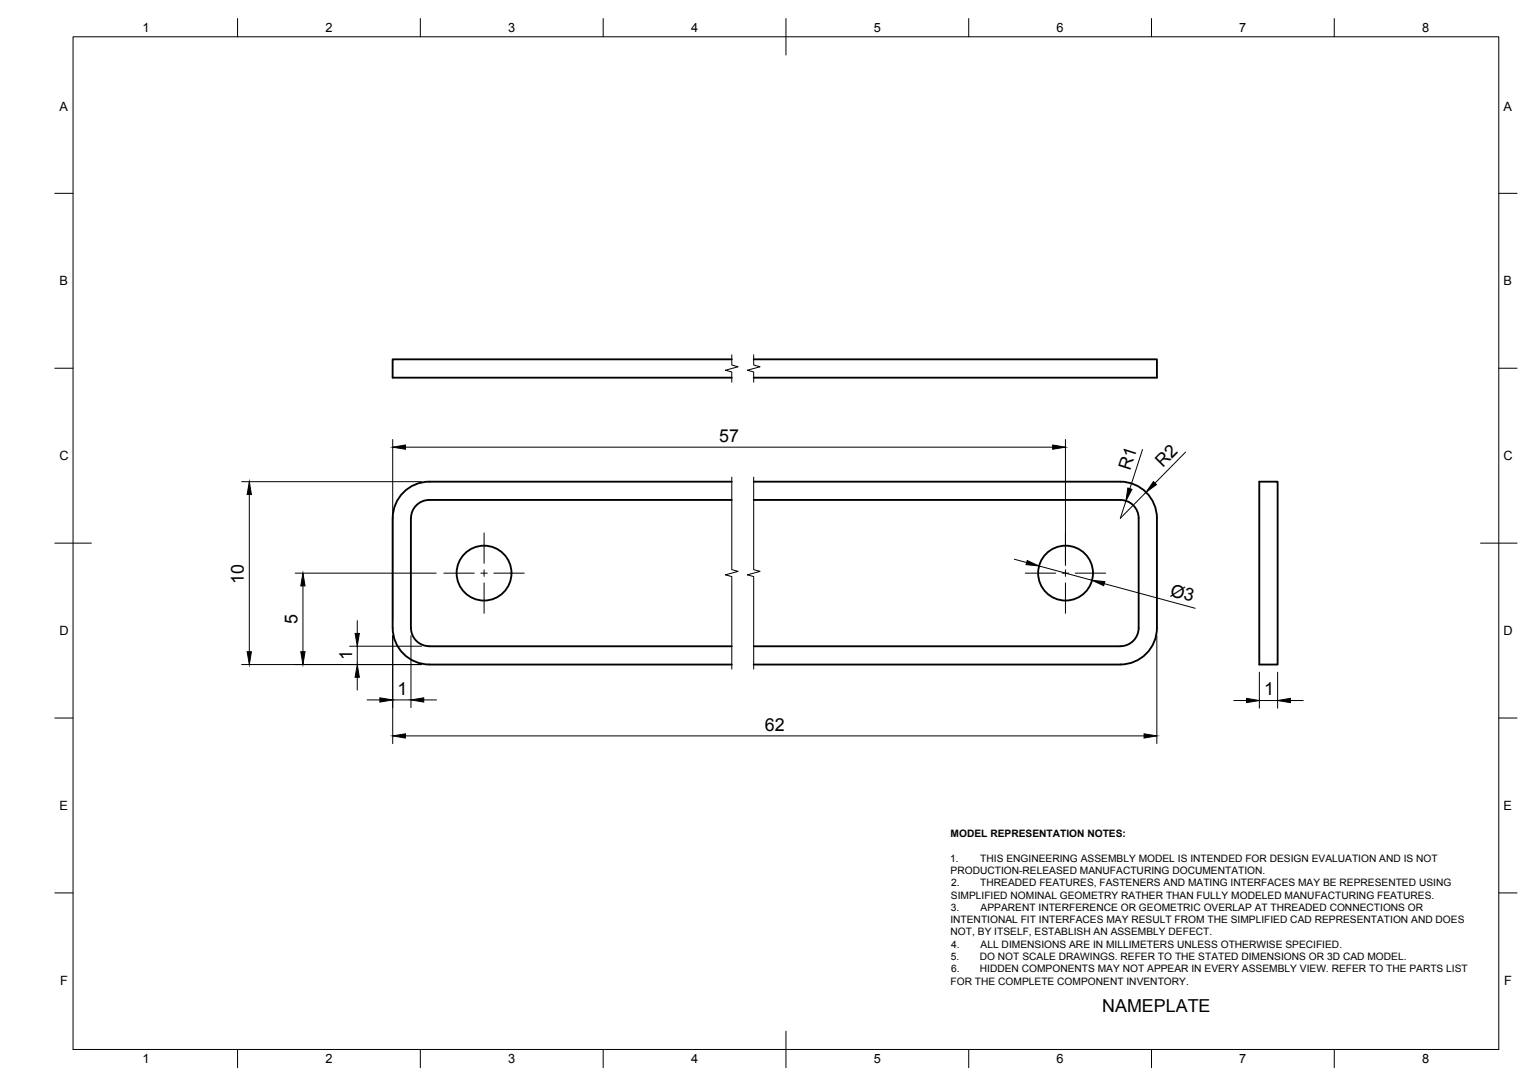
ISO-10303-21;
HEADER;
/* Generated by software containing ST-Developer
 * from STEP Tools, Inc. (www.steptools.com) 
 */

FILE_DESCRIPTION(
/* description */ (''),
/* implementation_level */ '2;1');

FILE_NAME(
/* name */ 'NAMEPLATE.step',
/* time_stamp */ '2026-10-06T01:16:10-07:00',
/* author */ (''),
/* organization */ (''),
/* preprocessor_version */ 'ST-DEVELOPER v20.2',
/* originating_system */ 'Autodesk Translation Framework v15.15.0.0',
/* authorisation */ '');

FILE_SCHEMA (('AUTOMOTIVE_DESIGN { 1 0 10303 214 3 1 1 }'));
ENDSEC;

DATA;
#10=MECHANICAL_DESIGN_GEOMETRIC_PRESENTATION_REPRESENTATION('',(#329),#17113);
#279=SHAPE_REPRESENTATION_RELATIONSHIP('SRR','None',#17205,#295);
#295=ADVANCED_BREP_SHAPE_REPRESENTATION('',(#345),#17112);
#329=STYLED_ITEM('',(#17298),#345);
#345=MANIFOLD_SOLID_BREP('Body1',#6031);
#494=CYLINDRICAL_SURFACE('',#6939,1.5);
#495=CYLINDRICAL_SURFACE('',#6947,1.);
#496=CYLINDRICAL_SURFACE('',#6957,2.);
#497=CYLINDRICAL_SURFACE('',#6959,2.);
#498=CYLINDRICAL_SURFACE('',#6961,2.);
#499=CYLINDRICAL_SURFACE('',#6963,2.);
#500=CYLINDRICAL_SURFACE('',#6966,1.);
#501=CYLINDRICAL_SURFACE('',#6968,1.);
#502=CYLINDRICAL_SURFACE('',#6970,1.);
#503=CYLINDRICAL_SURFACE('',#6972,1.5);
#631=FACE_BOUND('',#1835,.T.);
#632=FACE_BOUND('',#1836,.T.);
#633=FACE_BOUND('',#1839,.T.);
#634=FACE_BOUND('',#1840,.T.);
#635=FACE_BOUND('',#1843,.T.);
#988=CIRCLE('',#6933,2.);
#989=CIRCLE('',#6934,2.);
#990=CIRCLE('',#6935,2.);
#991=CIRCLE('',#6936,2.);
#992=CIRCLE('',#6937,1.5);
#993=CIRCLE('',#6938,1.5);
#994=CIRCLE('',#6940,1.5);
#995=CIRCLE('',#6942,1.);
#996=CIRCLE('',#6943,1.);
#997=CIRCLE('',#6944,1.);
#998=CIRCLE('',#6945,1.);
#999=CIRCLE('',#6946,1.5);
#1000=CIRCLE('',#6948,1.);
#1001=CIRCLE('',#6950,2.);
#1002=CIRCLE('',#6951,2.);
#1003=CIRCLE('',#6952,2.);
#1004=CIRCLE('',#6953,2.);
#1005=CIRCLE('',#6954,1.);
#1006=CIRCLE('',#6955,1.);
#1007=CIRCLE('',#6956,1.);
#1347=FACE_OUTER_BOUND('',#1834,.T.);
#1348=FACE_OUTER_BOUND('',#1837,.T.);
#1349=FACE_OUTER_BOUND('',#1838,.T.);
#1350=FACE_OUTER_BOUND('',#1841,.T.);
#1351=FACE_OUTER_BOUND('',#1842,.T.);
#1352=FACE_OUTER_BOUND('',#1844,.T.);
#1353=FACE_OUTER_BOUND('',#1845,.T.);
#1354=FACE_OUTER_BOUND('',#1846,.T.);
#1355=FACE_OUTER_BOUND('',#1847,.T.);
#1356=FACE_OUTER_BOUND('',#1848,.T.);
#1357=FACE_OUTER_BOUND('',#1849,.T.);
#1358=FACE_OUTER_BOUND('',#1850,.T.);
#1359=FACE_OUTER_BOUND('',#1851,.T.);
#1360=FACE_OUTER_BOUND('',#1852,.T.);
#1361=FACE_OUTER_BOUND('',#1853,.T.);
#1362=FACE_OUTER_BOUND('',#1854,.T.);
#1363=FACE_OUTER_BOUND('',#1855,.T.);
#1364=FACE_OUTER_BOUND('',#1856,.T.);
#1365=FACE_OUTER_BOUND('',#1857,.T.);
#1366=FACE_OUTER_BOUND('',#1858,.T.);
#1367=FACE_OUTER_BOUND('',#1859,.T.);
#1834=EDGE_LOOP('',(#5396,#5397,#5398,#5399,#5400,#5401,#5402,#5403));
#1835=EDGE_LOOP('',(#5404));
#1836=EDGE_LOOP('',(#5405));
#1837=EDGE_LOOP('',(#5406,#5407,#5408,#5409));
#1838=EDGE_LOOP('',(#5410,#5411,#5412,#5413,#5414,#5415,#5416,#5417));
#1839=EDGE_LOOP('',(#5418));
#1840=EDGE_LOOP('',(#5419));
#1841=EDGE_LOOP('',(#5420,#5421,#5422,#5423));
#1842=EDGE_LOOP('',(#5424,#5425,#5426,#5427,#5428,#5429,#5430,#5431));
#1843=EDGE_LOOP('',(#5432,#5433,#5434,#5435,#5436,#5437,#5438,#5439));
#1844=EDGE_LOOP('',(#5440,#5441,#5442,#5443));
#1845=EDGE_LOOP('',(#5444,#5445,#5446,#5447));
#1846=EDGE_LOOP('',(#5448,#5449,#5450,#5451));
#1847=EDGE_LOOP('',(#5452,#5453,#5454,#5455));
#1848=EDGE_LOOP('',(#5456,#5457,#5458,#5459));
#1849=EDGE_LOOP('',(#5460,#5461,#5462,#5463));
#1850=EDGE_LOOP('',(#5464,#5465,#5466,#5467));
#1851=EDGE_LOOP('',(#5468,#5469,#5470,#5471));
#1852=EDGE_LOOP('',(#5472,#5473,#5474,#5475));
#1853=EDGE_LOOP('',(#5476,#5477,#5478,#5479));
#1854=EDGE_LOOP('',(#5480,#5481,#5482,#5483));
#1855=EDGE_LOOP('',(#5484,#5485,#5486,#5487));
#1856=EDGE_LOOP('',(#5488,#5489,#5490,#5491));
#1857=EDGE_LOOP('',(#5492,#5493,#5494,#5495));
#1858=EDGE_LOOP('',(#5496,#5497,#5498,#5499));
#1859=EDGE_LOOP('',(#5500,#5501,#5502,#5503));
#2187=LINE('',#16957,#2548);
#2188=LINE('',#16961,#2549);
#2189=LINE('',#16965,#2550);
#2190=LINE('',#16968,#2551);
#2191=LINE('',#16975,#2552);
#2192=LINE('',#16982,#2553);
#2193=LINE('',#16986,#2554);
#2194=LINE('',#16990,#2555);
#2195=LINE('',#16993,#2556);
#2196=LINE('',#17000,#2557);
#2197=LINE('',#17001,#2558);
#2198=LINE('',#17007,#2559);
#2199=LINE('',#17011,#2560);
#2200=LINE('',#17015,#2561);
#2201=LINE('',#17018,#2562);
#2202=LINE('',#17020,#2563);
#2203=LINE('',#17024,#2564);
#2204=LINE('',#17028,#2565);
#2205=LINE('',#17031,#2566);
#2206=LINE('',#17033,#2567);
#2207=LINE('',#17034,#2568);
#2208=LINE('',#17036,#2569);
#2209=LINE('',#17038,#2570);
#2210=LINE('',#17040,#2571);
#2211=LINE('',#17042,#2572);
#2212=LINE('',#17044,#2573);
#2213=LINE('',#17046,#2574);
#2214=LINE('',#17049,#2575);
#2215=LINE('',#17051,#2576);
#2216=LINE('',#17053,#2577);
#2217=LINE('',#17055,#2578);
#2218=LINE('',#17057,#2579);
#2219=LINE('',#17059,#2580);
#2220=LINE('',#17062,#2581);
#2548=VECTOR('',#8755,58.);
#2549=VECTOR('',#8758,6.);
#2550=VECTOR('',#8761,58.);
#2551=VECTOR('',#8764,6.);
#2552=VECTOR('',#8771,1.5);
#2553=VECTOR('',#8778,6.);
#2554=VECTOR('',#8781,58.);
#2555=VECTOR('',#8784,6.);
#2556=VECTOR('',#8787,58.);
#2557=VECTOR('',#8794,0.5);
#2558=VECTOR('',#8795,0.5);
#2559=VECTOR('',#8800,6.);
#2560=VECTOR('',#8803,58.);
#2561=VECTOR('',#8806,6.);
#2562=VECTOR('',#8809,58.);
#2563=VECTOR('',#8810,58.);
#2564=VECTOR('',#8813,6.);
#2565=VECTOR('',#8816,58.);
#2566=VECTOR('',#8819,6.);
#2567=VECTOR('',#8822,1.);
#2568=VECTOR('',#8823,1.);
#2569=VECTOR('',#8826,1.);
#2570=VECTOR('',#8829,1.);
#2571=VECTOR('',#8832,1.);
#2572=VECTOR('',#8835,1.);
#2573=VECTOR('',#8838,1.);
#2574=VECTOR('',#8841,1.);
#2575=VECTOR('',#8846,0.5);
#2576=VECTOR('',#8849,0.5);
#2577=VECTOR('',#8852,0.5);
#2578=VECTOR('',#8855,0.5);
#2579=VECTOR('',#8858,0.5);
#2580=VECTOR('',#8861,0.5);
#2581=VECTOR('',#8866,1.5);
#3068=VERTEX_POINT('',#16953);
#3069=VERTEX_POINT('',#16954);
#3070=VERTEX_POINT('',#16956);
#3071=VERTEX_POINT('',#16958);
#3072=VERTEX_POINT('',#16960);
#3073=VERTEX_POINT('',#16962);
#3074=VERTEX_POINT('',#16964);
#3075=VERTEX_POINT('',#16966);
#3076=VERTEX_POINT('',#16969);
#3077=VERTEX_POINT('',#16971);
#3078=VERTEX_POINT('',#16974);
#3079=VERTEX_POINT('',#16978);
#3080=VERTEX_POINT('',#16979);
#3081=VERTEX_POINT('',#16981);
#3082=VERTEX_POINT('',#16983);
#3083=VERTEX_POINT('',#16985);
#3084=VERTEX_POINT('',#16987);
#3085=VERTEX_POINT('',#16989);
#3086=VERTEX_POINT('',#16991);
#3087=VERTEX_POINT('',#16994);
#3088=VERTEX_POINT('',#16997);
#3089=VERTEX_POINT('',#16998);
#3090=VERTEX_POINT('',#17003);
#3091=VERTEX_POINT('',#17004);
#3092=VERTEX_POINT('',#17006);
#3093=VERTEX_POINT('',#17008);
#3094=VERTEX_POINT('',#17010);
#3095=VERTEX_POINT('',#17012);
#3096=VERTEX_POINT('',#17014);
#3097=VERTEX_POINT('',#17016);
#3098=VERTEX_POINT('',#17019);
#3099=VERTEX_POINT('',#17021);
#3100=VERTEX_POINT('',#17023);
#3101=VERTEX_POINT('',#17025);
#3102=VERTEX_POINT('',#17027);
#3103=VERTEX_POINT('',#17029);
#3862=EDGE_CURVE('',#3068,#3069,#988,.T.);
#3863=EDGE_CURVE('',#3070,#3068,#2187,.T.);
#3864=EDGE_CURVE('',#3071,#3070,#989,.T.);
#3865=EDGE_CURVE('',#3072,#3071,#2188,.T.);
#3866=EDGE_CURVE('',#3073,#3072,#990,.T.);
#3867=EDGE_CURVE('',#3074,#3073,#2189,.T.);
#3868=EDGE_CURVE('',#3075,#3074,#991,.T.);
#3869=EDGE_CURVE('',#3069,#3075,#2190,.T.);
#3870=EDGE_CURVE('',#3076,#3076,#992,.T.);
#3871=EDGE_CURVE('',#3077,#3077,#993,.T.);
#3872=EDGE_CURVE('',#3077,#3078,#2191,.T.);
#3873=EDGE_CURVE('',#3078,#3078,#994,.T.);
#3874=EDGE_CURVE('',#3079,#3080,#995,.T.);
#3875=EDGE_CURVE('',#3080,#3081,#2192,.T.);
#3876=EDGE_CURVE('',#3081,#3082,#996,.T.);
#3877=EDGE_CURVE('',#3082,#3083,#2193,.T.);
#3878=EDGE_CURVE('',#3083,#3084,#997,.T.);
#3879=EDGE_CURVE('',#3084,#3085,#2194,.T.);
#3880=EDGE_CURVE('',#3085,#3086,#998,.T.);
#3881=EDGE_CURVE('',#3086,#3079,#2195,.T.);
#3882=EDGE_CURVE('',#3087,#3087,#999,.T.);
#3883=EDGE_CURVE('',#3088,#3089,#1000,.T.);
#3884=EDGE_CURVE('',#3089,#3080,#2196,.T.);
#3885=EDGE_CURVE('',#3088,#3079,#2197,.T.);
#3886=EDGE_CURVE('',#3090,#3091,#1001,.T.);
#3887=EDGE_CURVE('',#3091,#3092,#2198,.T.);
#3888=EDGE_CURVE('',#3092,#3093,#1002,.T.);
#3889=EDGE_CURVE('',#3093,#3094,#2199,.T.);
#3890=EDGE_CURVE('',#3094,#3095,#1003,.T.);
#3891=EDGE_CURVE('',#3095,#3096,#2200,.T.);
#3892=EDGE_CURVE('',#3096,#3097,#1004,.T.);
#3893=EDGE_CURVE('',#3097,#3090,#2201,.T.);
#3894=EDGE_CURVE('',#3098,#3088,#2202,.T.);
#3895=EDGE_CURVE('',#3099,#3098,#1005,.T.);
#3896=EDGE_CURVE('',#3100,#3099,#2203,.T.);
#3897=EDGE_CURVE('',#3101,#3100,#1006,.T.);
#3898=EDGE_CURVE('',#3102,#3101,#2204,.T.);
#3899=EDGE_CURVE('',#3103,#3102,#1007,.T.);
#3900=EDGE_CURVE('',#3089,#3103,#2205,.T.);
#3901=EDGE_CURVE('',#3069,#3091,#2206,.T.);
#3902=EDGE_CURVE('',#3068,#3090,#2207,.T.);
#3903=EDGE_CURVE('',#3070,#3097,#2208,.T.);
#3904=EDGE_CURVE('',#3071,#3096,#2209,.T.);
#3905=EDGE_CURVE('',#3072,#3095,#2210,.T.);
#3906=EDGE_CURVE('',#3073,#3094,#2211,.T.);
#3907=EDGE_CURVE('',#3074,#3093,#2212,.T.);
#3908=EDGE_CURVE('',#3075,#3092,#2213,.T.);
#3909=EDGE_CURVE('',#3103,#3081,#2214,.T.);
#3910=EDGE_CURVE('',#3102,#3082,#2215,.T.);
#3911=EDGE_CURVE('',#3101,#3083,#2216,.T.);
#3912=EDGE_CURVE('',#3100,#3084,#2217,.T.);
#3913=EDGE_CURVE('',#3099,#3085,#2218,.T.);
#3914=EDGE_CURVE('',#3098,#3086,#2219,.T.);
#3915=EDGE_CURVE('',#3076,#3087,#2220,.T.);
#5396=ORIENTED_EDGE('',*,*,#3862,.F.);
#5397=ORIENTED_EDGE('',*,*,#3863,.F.);
#5398=ORIENTED_EDGE('',*,*,#3864,.F.);
#5399=ORIENTED_EDGE('',*,*,#3865,.F.);
#5400=ORIENTED_EDGE('',*,*,#3866,.F.);
#5401=ORIENTED_EDGE('',*,*,#3867,.F.);
#5402=ORIENTED_EDGE('',*,*,#3868,.F.);
#5403=ORIENTED_EDGE('',*,*,#3869,.F.);
#5404=ORIENTED_EDGE('',*,*,#3870,.F.);
#5405=ORIENTED_EDGE('',*,*,#3871,.F.);
#5406=ORIENTED_EDGE('',*,*,#3871,.T.);
#5407=ORIENTED_EDGE('',*,*,#3872,.T.);
#5408=ORIENTED_EDGE('',*,*,#3873,.T.);
#5409=ORIENTED_EDGE('',*,*,#3872,.F.);
#5410=ORIENTED_EDGE('',*,*,#3874,.T.);
#5411=ORIENTED_EDGE('',*,*,#3875,.T.);
#5412=ORIENTED_EDGE('',*,*,#3876,.T.);
#5413=ORIENTED_EDGE('',*,*,#3877,.T.);
#5414=ORIENTED_EDGE('',*,*,#3878,.T.);
#5415=ORIENTED_EDGE('',*,*,#3879,.T.);
#5416=ORIENTED_EDGE('',*,*,#3880,.T.);
#5417=ORIENTED_EDGE('',*,*,#3881,.T.);
#5418=ORIENTED_EDGE('',*,*,#3873,.F.);
#5419=ORIENTED_EDGE('',*,*,#3882,.F.);
#5420=ORIENTED_EDGE('',*,*,#3883,.T.);
#5421=ORIENTED_EDGE('',*,*,#3884,.T.);
#5422=ORIENTED_EDGE('',*,*,#3874,.F.);
#5423=ORIENTED_EDGE('',*,*,#3885,.F.);
#5424=ORIENTED_EDGE('',*,*,#3886,.T.);
#5425=ORIENTED_EDGE('',*,*,#3887,.T.);
#5426=ORIENTED_EDGE('',*,*,#3888,.T.);
#5427=ORIENTED_EDGE('',*,*,#3889,.T.);
#5428=ORIENTED_EDGE('',*,*,#3890,.T.);
#5429=ORIENTED_EDGE('',*,*,#3891,.T.);
#5430=ORIENTED_EDGE('',*,*,#3892,.T.);
#5431=ORIENTED_EDGE('',*,*,#3893,.T.);
#5432=ORIENTED_EDGE('',*,*,#3883,.F.);
#5433=ORIENTED_EDGE('',*,*,#3894,.F.);
#5434=ORIENTED_EDGE('',*,*,#3895,.F.);
#5435=ORIENTED_EDGE('',*,*,#3896,.F.);
#5436=ORIENTED_EDGE('',*,*,#3897,.F.);
#5437=ORIENTED_EDGE('',*,*,#3898,.F.);
#5438=ORIENTED_EDGE('',*,*,#3899,.F.);
#5439=ORIENTED_EDGE('',*,*,#3900,.F.);
#5440=ORIENTED_EDGE('',*,*,#3862,.T.);
#5441=ORIENTED_EDGE('',*,*,#3901,.T.);
#5442=ORIENTED_EDGE('',*,*,#3886,.F.);
#5443=ORIENTED_EDGE('',*,*,#3902,.F.);
#5444=ORIENTED_EDGE('',*,*,#3863,.T.);
#5445=ORIENTED_EDGE('',*,*,#3902,.T.);
#5446=ORIENTED_EDGE('',*,*,#3893,.F.);
#5447=ORIENTED_EDGE('',*,*,#3903,.F.);
#5448=ORIENTED_EDGE('',*,*,#3864,.T.);
#5449=ORIENTED_EDGE('',*,*,#3903,.T.);
#5450=ORIENTED_EDGE('',*,*,#3892,.F.);
#5451=ORIENTED_EDGE('',*,*,#3904,.F.);
#5452=ORIENTED_EDGE('',*,*,#3865,.T.);
#5453=ORIENTED_EDGE('',*,*,#3904,.T.);
#5454=ORIENTED_EDGE('',*,*,#3891,.F.);
#5455=ORIENTED_EDGE('',*,*,#3905,.F.);
#5456=ORIENTED_EDGE('',*,*,#3866,.T.);
#5457=ORIENTED_EDGE('',*,*,#3905,.T.);
#5458=ORIENTED_EDGE('',*,*,#3890,.F.);
#5459=ORIENTED_EDGE('',*,*,#3906,.F.);
#5460=ORIENTED_EDGE('',*,*,#3867,.T.);
#5461=ORIENTED_EDGE('',*,*,#3906,.T.);
#5462=ORIENTED_EDGE('',*,*,#3889,.F.);
#5463=ORIENTED_EDGE('',*,*,#3907,.F.);
#5464=ORIENTED_EDGE('',*,*,#3868,.T.);
#5465=ORIENTED_EDGE('',*,*,#3907,.T.);
#5466=ORIENTED_EDGE('',*,*,#3888,.F.);
#5467=ORIENTED_EDGE('',*,*,#3908,.F.);
#5468=ORIENTED_EDGE('',*,*,#3869,.T.);
#5469=ORIENTED_EDGE('',*,*,#3908,.T.);
#5470=ORIENTED_EDGE('',*,*,#3887,.F.);
#5471=ORIENTED_EDGE('',*,*,#3901,.F.);
#5472=ORIENTED_EDGE('',*,*,#3900,.T.);
#5473=ORIENTED_EDGE('',*,*,#3909,.T.);
#5474=ORIENTED_EDGE('',*,*,#3875,.F.);
#5475=ORIENTED_EDGE('',*,*,#3884,.F.);
#5476=ORIENTED_EDGE('',*,*,#3899,.T.);
#5477=ORIENTED_EDGE('',*,*,#3910,.T.);
#5478=ORIENTED_EDGE('',*,*,#3876,.F.);
#5479=ORIENTED_EDGE('',*,*,#3909,.F.);
#5480=ORIENTED_EDGE('',*,*,#3898,.T.);
#5481=ORIENTED_EDGE('',*,*,#3911,.T.);
#5482=ORIENTED_EDGE('',*,*,#3877,.F.);
#5483=ORIENTED_EDGE('',*,*,#3910,.F.);
#5484=ORIENTED_EDGE('',*,*,#3897,.T.);
#5485=ORIENTED_EDGE('',*,*,#3912,.T.);
#5486=ORIENTED_EDGE('',*,*,#3878,.F.);
#5487=ORIENTED_EDGE('',*,*,#3911,.F.);
#5488=ORIENTED_EDGE('',*,*,#3896,.T.);
#5489=ORIENTED_EDGE('',*,*,#3913,.T.);
#5490=ORIENTED_EDGE('',*,*,#3879,.F.);
#5491=ORIENTED_EDGE('',*,*,#3912,.F.);
#5492=ORIENTED_EDGE('',*,*,#3895,.T.);
#5493=ORIENTED_EDGE('',*,*,#3914,.T.);
#5494=ORIENTED_EDGE('',*,*,#3880,.F.);
#5495=ORIENTED_EDGE('',*,*,#3913,.F.);
#5496=ORIENTED_EDGE('',*,*,#3894,.T.);
#5497=ORIENTED_EDGE('',*,*,#3885,.T.);
#5498=ORIENTED_EDGE('',*,*,#3881,.F.);
#5499=ORIENTED_EDGE('',*,*,#3914,.F.);
#5500=ORIENTED_EDGE('',*,*,#3870,.T.);
#5501=ORIENTED_EDGE('',*,*,#3915,.T.);
#5502=ORIENTED_EDGE('',*,*,#3882,.T.);
#5503=ORIENTED_EDGE('',*,*,#3915,.F.);
#5645=PLANE('',#6932);
#5646=PLANE('',#6941);
#5647=PLANE('',#6949);
#5648=PLANE('',#6958);
#5649=PLANE('',#6960);
#5650=PLANE('',#6962);
#5651=PLANE('',#6964);
#5652=PLANE('',#6965);
#5653=PLANE('',#6967);
#5654=PLANE('',#6969);
#5655=PLANE('',#6971);
#5995=ADVANCED_FACE('',(#1347,#631,#632),#5645,.F.);
#5996=ADVANCED_FACE('',(#1348),#494,.F.);
#5997=ADVANCED_FACE('',(#1349,#633,#634),#5646,.T.);
#5998=ADVANCED_FACE('',(#1350),#495,.F.);
#5999=ADVANCED_FACE('',(#1351,#635),#5647,.T.);
#6000=ADVANCED_FACE('',(#1352),#496,.T.);
#6001=ADVANCED_FACE('',(#1353),#5648,.T.);
#6002=ADVANCED_FACE('',(#1354),#497,.T.);
#6003=ADVANCED_FACE('',(#1355),#5649,.T.);
#6004=ADVANCED_FACE('',(#1356),#498,.T.);
#6005=ADVANCED_FACE('',(#1357),#5650,.T.);
#6006=ADVANCED_FACE('',(#1358),#499,.T.);
#6007=ADVANCED_FACE('',(#1359),#5651,.T.);
#6008=ADVANCED_FACE('',(#1360),#5652,.F.);
#6009=ADVANCED_FACE('',(#1361),#500,.F.);
#6010=ADVANCED_FACE('',(#1362),#5653,.F.);
#6011=ADVANCED_FACE('',(#1363),#501,.F.);
#6012=ADVANCED_FACE('',(#1364),#5654,.F.);
#6013=ADVANCED_FACE('',(#1365),#502,.F.);
#6014=ADVANCED_FACE('',(#1366),#5655,.F.);
#6015=ADVANCED_FACE('',(#1367),#503,.F.);
#6031=CLOSED_SHELL('',(#5995,#5996,#5997,#5998,#5999,#6000,#6001,#6002,
#6003,#6004,#6005,#6006,#6007,#6008,#6009,#6010,#6011,#6012,#6013,#6014,
#6015));
#6931=AXIS2_PLACEMENT_3D('',#16951,#8749,#8750);
#6932=AXIS2_PLACEMENT_3D('',#16952,#8751,#8752);
#6933=AXIS2_PLACEMENT_3D('',#16955,#8753,#8754);
#6934=AXIS2_PLACEMENT_3D('',#16959,#8756,#8757);
#6935=AXIS2_PLACEMENT_3D('',#16963,#8759,#8760);
#6936=AXIS2_PLACEMENT_3D('',#16967,#8762,#8763);
#6937=AXIS2_PLACEMENT_3D('',#16970,#8765,#8766);
#6938=AXIS2_PLACEMENT_3D('',#16972,#8767,#8768);
#6939=AXIS2_PLACEMENT_3D('',#16973,#8769,#8770);
#6940=AXIS2_PLACEMENT_3D('',#16976,#8772,#8773);
#6941=AXIS2_PLACEMENT_3D('',#16977,#8774,#8775);
#6942=AXIS2_PLACEMENT_3D('',#16980,#8776,#8777);
#6943=AXIS2_PLACEMENT_3D('',#16984,#8779,#8780);
#6944=AXIS2_PLACEMENT_3D('',#16988,#8782,#8783);
#6945=AXIS2_PLACEMENT_3D('',#16992,#8785,#8786);
#6946=AXIS2_PLACEMENT_3D('',#16995,#8788,#8789);
#6947=AXIS2_PLACEMENT_3D('',#16996,#8790,#8791);
#6948=AXIS2_PLACEMENT_3D('',#16999,#8792,#8793);
#6949=AXIS2_PLACEMENT_3D('',#17002,#8796,#8797);
#6950=AXIS2_PLACEMENT_3D('',#17005,#8798,#8799);
#6951=AXIS2_PLACEMENT_3D('',#17009,#8801,#8802);
#6952=AXIS2_PLACEMENT_3D('',#17013,#8804,#8805);
#6953=AXIS2_PLACEMENT_3D('',#17017,#8807,#8808);
#6954=AXIS2_PLACEMENT_3D('',#17022,#8811,#8812);
#6955=AXIS2_PLACEMENT_3D('',#17026,#8814,#8815);
#6956=AXIS2_PLACEMENT_3D('',#17030,#8817,#8818);
#6957=AXIS2_PLACEMENT_3D('',#17032,#8820,#8821);
#6958=AXIS2_PLACEMENT_3D('',#17035,#8824,#8825);
#6959=AXIS2_PLACEMENT_3D('',#17037,#8827,#8828);
#6960=AXIS2_PLACEMENT_3D('',#17039,#8830,#8831);
#6961=AXIS2_PLACEMENT_3D('',#17041,#8833,#8834);
#6962=AXIS2_PLACEMENT_3D('',#17043,#8836,#8837);
#6963=AXIS2_PLACEMENT_3D('',#17045,#8839,#8840);
#6964=AXIS2_PLACEMENT_3D('',#17047,#8842,#8843);
#6965=AXIS2_PLACEMENT_3D('',#17048,#8844,#8845);
#6966=AXIS2_PLACEMENT_3D('',#17050,#8847,#8848);
#6967=AXIS2_PLACEMENT_3D('',#17052,#8850,#8851);
#6968=AXIS2_PLACEMENT_3D('',#17054,#8853,#8854);
#6969=AXIS2_PLACEMENT_3D('',#17056,#8856,#8857);
#6970=AXIS2_PLACEMENT_3D('',#17058,#8859,#8860);
#6971=AXIS2_PLACEMENT_3D('',#17060,#8862,#8863);
#6972=AXIS2_PLACEMENT_3D('',#17061,#8864,#8865);
#8749=DIRECTION('axis',(0.,0.,1.));
#8750=DIRECTION('refdir',(1.,0.,0.));
#8751=DIRECTION('center_axis',(0.,0.,1.));
#8752=DIRECTION('ref_axis',(1.,0.,0.));
#8753=DIRECTION('center_axis',(0.,0.,1.));
#8754=DIRECTION('ref_axis',(0.,1.,0.));
#8755=DIRECTION('',(-1.,0.,0.));
#8756=DIRECTION('center_axis',(0.,0.,1.));
#8757=DIRECTION('ref_axis',(1.,0.,0.));
#8758=DIRECTION('',(0.,1.,0.));
#8759=DIRECTION('center_axis',(0.,0.,1.));
#8760=DIRECTION('ref_axis',(0.,-1.,0.));
#8761=DIRECTION('',(1.,0.,0.));
#8762=DIRECTION('center_axis',(0.,0.,1.));
#8763=DIRECTION('ref_axis',(-1.,0.,0.));
#8764=DIRECTION('',(0.,-1.,0.));
#8765=DIRECTION('center_axis',(0.,0.,-1.));
#8766=DIRECTION('ref_axis',(1.,0.,0.));
#8767=DIRECTION('center_axis',(0.,0.,-1.));
#8768=DIRECTION('ref_axis',(1.,0.,0.));
#8769=DIRECTION('center_axis',(0.,0.,1.));
#8770=DIRECTION('ref_axis',(1.,0.,0.));
#8771=DIRECTION('',(0.,0.,1.));
#8772=DIRECTION('center_axis',(0.,0.,1.));
#8773=DIRECTION('ref_axis',(-1.,0.,0.));
#8774=DIRECTION('center_axis',(0.,0.,1.));
#8775=DIRECTION('ref_axis',(1.,0.,0.));
#8776=DIRECTION('center_axis',(0.,0.,1.));
#8777=DIRECTION('ref_axis',(0.,1.,0.));
#8778=DIRECTION('',(0.,-1.,0.));
#8779=DIRECTION('center_axis',(0.,0.,1.));
#8780=DIRECTION('ref_axis',(-1.,0.,0.));
#8781=DIRECTION('',(1.,0.,0.));
#8782=DIRECTION('center_axis',(0.,0.,1.));
#8783=DIRECTION('ref_axis',(0.,-1.,0.));
#8784=DIRECTION('',(0.,1.,0.));
#8785=DIRECTION('center_axis',(0.,0.,1.));
#8786=DIRECTION('ref_axis',(1.,0.,0.));
#8787=DIRECTION('',(-1.,0.,0.));
#8788=DIRECTION('center_axis',(0.,0.,1.));
#8789=DIRECTION('ref_axis',(-1.,0.,0.));
#8790=DIRECTION('center_axis',(0.,0.,1.));
#8791=DIRECTION('ref_axis',(1.,0.,0.));
#8792=DIRECTION('center_axis',(0.,0.,1.));
#8793=DIRECTION('ref_axis',(0.,1.,0.));
#8794=DIRECTION('',(0.,0.,-1.));
#8795=DIRECTION('',(0.,0.,-1.));
#8796=DIRECTION('center_axis',(0.,0.,1.));
#8797=DIRECTION('ref_axis',(1.,0.,0.));
#8798=DIRECTION('center_axis',(0.,0.,1.));
#8799=DIRECTION('ref_axis',(0.,1.,0.));
#8800=DIRECTION('',(0.,-1.,0.));
#8801=DIRECTION('center_axis',(0.,0.,1.));
#8802=DIRECTION('ref_axis',(-1.,0.,0.));
#8803=DIRECTION('',(1.,0.,0.));
#8804=DIRECTION('center_axis',(0.,0.,1.));
#8805=DIRECTION('ref_axis',(0.,-1.,0.));
#8806=DIRECTION('',(0.,1.,0.));
#8807=DIRECTION('center_axis',(0.,0.,1.));
#8808=DIRECTION('ref_axis',(1.,0.,0.));
#8809=DIRECTION('',(-1.,0.,0.));
#8810=DIRECTION('',(-1.,0.,0.));
#8811=DIRECTION('center_axis',(0.,0.,1.));
#8812=DIRECTION('ref_axis',(1.,0.,0.));
#8813=DIRECTION('',(0.,1.,0.));
#8814=DIRECTION('center_axis',(0.,0.,1.));
#8815=DIRECTION('ref_axis',(0.,-1.,0.));
#8816=DIRECTION('',(1.,0.,0.));
#8817=DIRECTION('center_axis',(0.,0.,1.));
#8818=DIRECTION('ref_axis',(-1.,0.,0.));
#8819=DIRECTION('',(0.,-1.,0.));
#8820=DIRECTION('center_axis',(0.,0.,1.));
#8821=DIRECTION('ref_axis',(1.,0.,0.));
#8822=DIRECTION('',(0.,0.,1.));
#8823=DIRECTION('',(0.,0.,1.));
#8824=DIRECTION('center_axis',(0.,1.,0.));
#8825=DIRECTION('ref_axis',(-1.,0.,0.));
#8826=DIRECTION('',(0.,0.,1.));
#8827=DIRECTION('center_axis',(0.,0.,1.));
#8828=DIRECTION('ref_axis',(1.,0.,0.));
#8829=DIRECTION('',(0.,0.,1.));
#8830=DIRECTION('center_axis',(1.,0.,0.));
#8831=DIRECTION('ref_axis',(0.,1.,0.));
#8832=DIRECTION('',(0.,0.,1.));
#8833=DIRECTION('center_axis',(0.,0.,1.));
#8834=DIRECTION('ref_axis',(1.,0.,0.));
#8835=DIRECTION('',(0.,0.,1.));
#8836=DIRECTION('center_axis',(0.,-1.,0.));
#8837=DIRECTION('ref_axis',(1.,0.,0.));
#8838=DIRECTION('',(0.,0.,1.));
#8839=DIRECTION('center_axis',(0.,0.,1.));
#8840=DIRECTION('ref_axis',(1.,0.,0.));
#8841=DIRECTION('',(0.,0.,1.));
#8842=DIRECTION('center_axis',(-1.,0.,0.));
#8843=DIRECTION('ref_axis',(0.,-1.,0.));
#8844=DIRECTION('center_axis',(-1.,0.,0.));
#8845=DIRECTION('ref_axis',(0.,-1.,0.));
#8846=DIRECTION('',(0.,0.,-1.));
#8847=DIRECTION('center_axis',(0.,0.,1.));
#8848=DIRECTION('ref_axis',(1.,0.,0.));
#8849=DIRECTION('',(0.,0.,-1.));
#8850=DIRECTION('center_axis',(0.,-1.,0.));
#8851=DIRECTION('ref_axis',(1.,0.,0.));
#8852=DIRECTION('',(0.,0.,-1.));
#8853=DIRECTION('center_axis',(0.,0.,1.));
#8854=DIRECTION('ref_axis',(1.,0.,0.));
#8855=DIRECTION('',(0.,0.,-1.));
#8856=DIRECTION('center_axis',(1.,0.,0.));
#8857=DIRECTION('ref_axis',(0.,1.,0.));
#8858=DIRECTION('',(0.,0.,-1.));
#8859=DIRECTION('center_axis',(0.,0.,1.));
#8860=DIRECTION('ref_axis',(1.,0.,0.));
#8861=DIRECTION('',(0.,0.,-1.));
#8862=DIRECTION('center_axis',(0.,1.,0.));
#8863=DIRECTION('ref_axis',(-1.,0.,0.));
#8864=DIRECTION('center_axis',(0.,0.,1.));
#8865=DIRECTION('ref_axis',(1.,0.,0.));
#8866=DIRECTION('',(0.,0.,1.));
#16951=CARTESIAN_POINT('',(0.,0.,0.));
#16952=CARTESIAN_POINT('Origin',(0.,0.,-0.5));
#16953=CARTESIAN_POINT('',(-29.,5.,-0.5));
#16954=CARTESIAN_POINT('',(-31.,3.,-0.5));
#16955=CARTESIAN_POINT('Origin',(-29.,3.,-0.5));
#16956=CARTESIAN_POINT('',(29.,5.,-0.5));
#16957=CARTESIAN_POINT('',(29.,5.,-0.5));
#16958=CARTESIAN_POINT('',(31.,3.,-0.5));
#16959=CARTESIAN_POINT('Origin',(29.,3.,-0.5));
#16960=CARTESIAN_POINT('',(31.,-3.,-0.5));
#16961=CARTESIAN_POINT('',(31.,-3.,-0.5));
#16962=CARTESIAN_POINT('',(29.,-5.,-0.5));
#16963=CARTESIAN_POINT('Origin',(29.,-3.,-0.5));
#16964=CARTESIAN_POINT('',(-29.,-5.,-0.5));
#16965=CARTESIAN_POINT('',(-29.,-5.,-0.5));
#16966=CARTESIAN_POINT('',(-31.,-3.,-0.5));
#16967=CARTESIAN_POINT('Origin',(-29.,-3.,-0.5));
#16968=CARTESIAN_POINT('',(-31.,3.,-0.5));
#16969=CARTESIAN_POINT('',(24.5,0.,-0.5));
#16970=CARTESIAN_POINT('Origin',(26.,0.,-0.5));
#16971=CARTESIAN_POINT('',(-27.5,0.,-0.5));
#16972=CARTESIAN_POINT('Origin',(-26.,0.,-0.5));
#16973=CARTESIAN_POINT('Origin',(-26.,0.,-0.5));
#16974=CARTESIAN_POINT('',(-27.5,0.,0.));
#16975=CARTESIAN_POINT('',(-27.5,-1.83697019872103E-16,-0.5));
#16976=CARTESIAN_POINT('Origin',(-26.,0.,0.));
#16977=CARTESIAN_POINT('Origin',(0.,0.,0.));
#16978=CARTESIAN_POINT('',(-29.,4.,0.));
#16979=CARTESIAN_POINT('',(-30.,3.,0.));
#16980=CARTESIAN_POINT('Origin',(-29.,3.,0.));
#16981=CARTESIAN_POINT('',(-30.,-3.,0.));
#16982=CARTESIAN_POINT('',(-30.,3.,0.));
#16983=CARTESIAN_POINT('',(-29.,-4.,0.));
#16984=CARTESIAN_POINT('Origin',(-29.,-3.,0.));
#16985=CARTESIAN_POINT('',(29.,-4.,0.));
#16986=CARTESIAN_POINT('',(-29.,-4.,0.));
#16987=CARTESIAN_POINT('',(30.,-3.,0.));
#16988=CARTESIAN_POINT('Origin',(29.,-3.,0.));
#16989=CARTESIAN_POINT('',(30.,3.,0.));
#16990=CARTESIAN_POINT('',(30.,-3.,0.));
#16991=CARTESIAN_POINT('',(29.,4.,0.));
#16992=CARTESIAN_POINT('Origin',(29.,3.,0.));
#16993=CARTESIAN_POINT('',(29.,4.,0.));
#16994=CARTESIAN_POINT('',(24.5,0.,0.));
#16995=CARTESIAN_POINT('Origin',(26.,0.,0.));
#16996=CARTESIAN_POINT('Origin',(-29.,3.,0.5));
#16997=CARTESIAN_POINT('',(-29.,4.,0.5));
#16998=CARTESIAN_POINT('',(-30.,3.,0.5));
#16999=CARTESIAN_POINT('Origin',(-29.,3.,0.5));
#17000=CARTESIAN_POINT('',(-30.,3.,0.5));
#17001=CARTESIAN_POINT('',(-29.,4.,0.5));
#17002=CARTESIAN_POINT('Origin',(0.,0.,0.5));
#17003=CARTESIAN_POINT('',(-29.,5.,0.5));
#17004=CARTESIAN_POINT('',(-31.,3.,0.5));
#17005=CARTESIAN_POINT('Origin',(-29.,3.,0.5));
#17006=CARTESIAN_POINT('',(-31.,-3.,0.5));
#17007=CARTESIAN_POINT('',(-31.,3.,0.5));
#17008=CARTESIAN_POINT('',(-29.,-5.,0.5));
#17009=CARTESIAN_POINT('Origin',(-29.,-3.,0.5));
#17010=CARTESIAN_POINT('',(29.,-5.,0.5));
#17011=CARTESIAN_POINT('',(-29.,-5.,0.5));
#17012=CARTESIAN_POINT('',(31.,-3.,0.5));
#17013=CARTESIAN_POINT('Origin',(29.,-3.,0.5));
#17014=CARTESIAN_POINT('',(31.,3.,0.5));
#17015=CARTESIAN_POINT('',(31.,-3.,0.5));
#17016=CARTESIAN_POINT('',(29.,5.,0.5));
#17017=CARTESIAN_POINT('Origin',(29.,3.,0.5));
#17018=CARTESIAN_POINT('',(29.,5.,0.5));
#17019=CARTESIAN_POINT('',(29.,4.,0.5));
#17020=CARTESIAN_POINT('',(29.,4.,0.5));
#17021=CARTESIAN_POINT('',(30.,3.,0.5));
#17022=CARTESIAN_POINT('Origin',(29.,3.,0.5));
#17023=CARTESIAN_POINT('',(30.,-3.,0.5));
#17024=CARTESIAN_POINT('',(30.,-3.,0.5));
#17025=CARTESIAN_POINT('',(29.,-4.,0.5));
#17026=CARTESIAN_POINT('Origin',(29.,-3.,0.5));
#17027=CARTESIAN_POINT('',(-29.,-4.,0.5));
#17028=CARTESIAN_POINT('',(-29.,-4.,0.5));
#17029=CARTESIAN_POINT('',(-30.,-3.,0.5));
#17030=CARTESIAN_POINT('Origin',(-29.,-3.,0.5));
#17031=CARTESIAN_POINT('',(-30.,3.,0.5));
#17032=CARTESIAN_POINT('Origin',(-29.,3.,-0.5));
#17033=CARTESIAN_POINT('',(-31.,3.,-0.5));
#17034=CARTESIAN_POINT('',(-29.,5.,-0.5));
#17035=CARTESIAN_POINT('Origin',(29.,5.,-0.5));
#17036=CARTESIAN_POINT('',(29.,5.,-0.5));
#17037=CARTESIAN_POINT('Origin',(29.,3.,-0.5));
#17038=CARTESIAN_POINT('',(31.,3.,-0.5));
#17039=CARTESIAN_POINT('Origin',(31.,-3.,-0.5));
#17040=CARTESIAN_POINT('',(31.,-3.,-0.5));
#17041=CARTESIAN_POINT('Origin',(29.,-3.,-0.5));
#17042=CARTESIAN_POINT('',(29.,-5.,-0.5));
#17043=CARTESIAN_POINT('Origin',(-29.,-5.,-0.5));
#17044=CARTESIAN_POINT('',(-29.,-5.,-0.5));
#17045=CARTESIAN_POINT('Origin',(-29.,-3.,-0.5));
#17046=CARTESIAN_POINT('',(-31.,-3.,-0.5));
#17047=CARTESIAN_POINT('Origin',(-31.,3.,-0.5));
#17048=CARTESIAN_POINT('Origin',(-30.,3.,0.5));
#17049=CARTESIAN_POINT('',(-30.,-3.,0.5));
#17050=CARTESIAN_POINT('Origin',(-29.,-3.,0.5));
#17051=CARTESIAN_POINT('',(-29.,-4.,0.5));
#17052=CARTESIAN_POINT('Origin',(-29.,-4.,0.5));
#17053=CARTESIAN_POINT('',(29.,-4.,0.5));
#17054=CARTESIAN_POINT('Origin',(29.,-3.,0.5));
#17055=CARTESIAN_POINT('',(30.,-3.,0.5));
#17056=CARTESIAN_POINT('Origin',(30.,-3.,0.5));
#17057=CARTESIAN_POINT('',(30.,3.,0.5));
#17058=CARTESIAN_POINT('Origin',(29.,3.,0.5));
#17059=CARTESIAN_POINT('',(29.,4.,0.5));
#17060=CARTESIAN_POINT('Origin',(29.,4.,0.5));
#17061=CARTESIAN_POINT('Origin',(26.,0.,-0.5));
#17062=CARTESIAN_POINT('',(24.5,-1.83697019872103E-16,-0.5));
#17089=UNCERTAINTY_MEASURE_WITH_UNIT(LENGTH_MEASURE(0.01),#17114,
'DISTANCE_ACCURACY_VALUE',
'Maximum model space distance between geometric entities at asserted c
onnectivities');
#17090=UNCERTAINTY_MEASURE_WITH_UNIT(LENGTH_MEASURE(0.01),#17114,
'DISTANCE_ACCURACY_VALUE',
'Maximum model space distance between geometric entities at asserted c
onnectivities');
#17112=(
GEOMETRIC_REPRESENTATION_CONTEXT(3)
GLOBAL_UNCERTAINTY_ASSIGNED_CONTEXT((#17089))
GLOBAL_UNIT_ASSIGNED_CONTEXT((#17114,#17116,#17117))
REPRESENTATION_CONTEXT('','3D')
);
#17113=(
GEOMETRIC_REPRESENTATION_CONTEXT(3)
GLOBAL_UNCERTAINTY_ASSIGNED_CONTEXT((#17090))
GLOBAL_UNIT_ASSIGNED_CONTEXT((#17114,#17116,#17117))
REPRESENTATION_CONTEXT('','3D')
);
#17114=(
LENGTH_UNIT()
NAMED_UNIT(*)
SI_UNIT(.MILLI.,.METRE.)
);
#17116=(
NAMED_UNIT(*)
PLANE_ANGLE_UNIT()
SI_UNIT($,.RADIAN.)
);
#17117=(
NAMED_UNIT(*)
SI_UNIT($,.STERADIAN.)
SOLID_ANGLE_UNIT()
);
#17139=SHAPE_DEFINITION_REPRESENTATION(#17178,#17205);
#17178=PRODUCT_DEFINITION_SHAPE('',$,#17228);
#17205=SHAPE_REPRESENTATION('',(#6931),#17112);
#17206=PRODUCT_DEFINITION_CONTEXT('part definition',#17274,'design');
#17228=PRODUCT_DEFINITION('NAMEPLATE','NAMEPLATE',#17250,#17206);
#17250=PRODUCT_DEFINITION_FORMATION('',$,#17297);
#17274=APPLICATION_CONTEXT(
'Core Data for Automotive Mechanical Design Process');
#17275=PRODUCT_CONTEXT('part definition',#17274,'mechanical');
#17297=PRODUCT('NAMEPLATE','NAMEPLATE','NOT SPECIFIED',(#17275));
#17298=PRESENTATION_STYLE_ASSIGNMENT((#17299));
#17299=SURFACE_STYLE_USAGE(.BOTH.,#17300);
#17300=SURFACE_SIDE_STYLE('',(#17301));
#17301=SURFACE_STYLE_FILL_AREA(#17302);
#17302=FILL_AREA_STYLE('Steel - Satin',(#17303));
#17303=FILL_AREA_STYLE_COLOUR('Steel - Satin',#17304);
#17304=COLOUR_RGB('Steel - Satin', 0.09019608, 0.27058824, 0.51372549);
ENDSEC;
END-ISO-10303-21;
